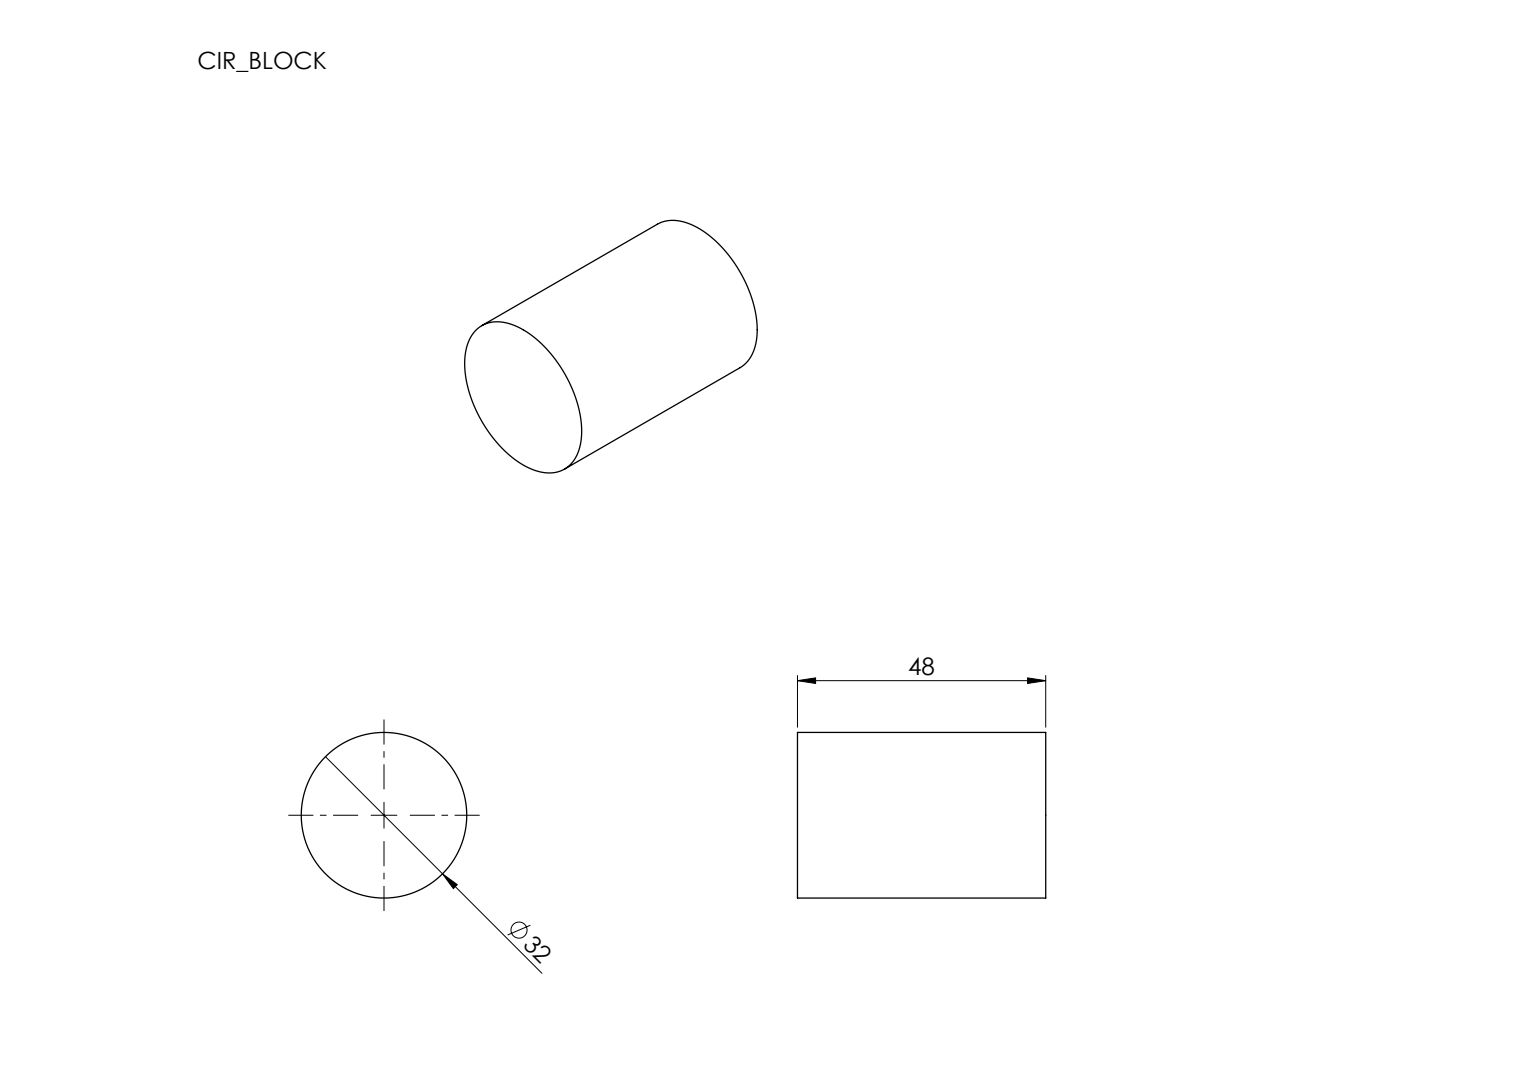
ISO-10303-21;
HEADER;
FILE_DESCRIPTION (('STEP AP214'),
    '1' );
FILE_NAME ('cir_block.step',
    '2026-10-08T13:22:57',
    ( '' ),
    ( '' ),
    'SwSTEP 2.0',
    'SolidWorks 2026',
    '' );
FILE_SCHEMA (( 'AUTOMOTIVE_DESIGN' ));
ENDSEC;

DATA;
#31=CARTESIAN_POINT ( 'NONE',  ( 0.000000000000000000, -6.162975822039154730E-30, 20.00000000000001776 ) ) ;
#245=CARTESIAN_POINT ( 'NONE',  ( 0.000000000000000000, 0.000000000000000000, 0.000000000000000000 ) ) ;
#365=( LENGTH_UNIT ( ) NAMED_UNIT ( * ) SI_UNIT ( .MILLI., .METRE. ) );
#415=( NAMED_UNIT ( * ) SI_UNIT ( $, .STERADIAN. ) SOLID_ANGLE_UNIT ( ) );
#499=AXIS2_PLACEMENT_3D ( 'NONE', #9498, #7831, #2505 ) ;
#736=DIRECTION ( 'NONE',  ( 0.000000000000000000, 0.000000000000000000, 1.000000000000000000 ) ) ;
#821=ORIENTED_EDGE ( 'NONE', *, *, #1366, .T. ) ;
#931=CYLINDRICAL_SURFACE ( 'NONE', #9784, 16.00000000000000000 ) ;
#1013=AXIS2_PLACEMENT_3D ( 'NONE', #4039, #3151, #6292 ) ;
#1129=ORIENTED_EDGE ( 'NONE', *, *, #9823, .F. ) ;
#1366=EDGE_CURVE ( 'NONE', #7651, #3104, #9591, .T. ) ;
#1410=SURFACE_SIDE_STYLE ('',( #7076 ) ) ;
#1441=COLOUR_RGB ( '', 0.08235294, 0.09019608, 0.10196078) ;
#1635=EDGE_LOOP ( 'NONE', ( #7592, #4013, #4601, #9629 ) ) ;
#1651=VERTEX_POINT ( 'NONE', #9037 ) ;
#1743=UNCERTAINTY_MEASURE_WITH_UNIT (LENGTH_MEASURE( 1.000000000000000082E-05 ), #365, 'distance_accuracy_value', 'NONE');
#1806=ADVANCED_FACE ( 'NONE', ( #7936 ), #3077, .F. ) ;
#1865=VECTOR ( 'NONE', #9017, 1000.000000000000000 ) ;
#1959=ORIENTED_EDGE ( 'NONE', *, *, #1366, .F. ) ;
#2023=CARTESIAN_POINT ( 'NONE',  ( 0.000000000000000000, -6.162975822039154730E-30, 20.00000000000001776 ) ) ;
#2058=PRODUCT_CONTEXT ( 'NONE', #2562, 'mechanical' ) ;
#2064=PRESENTATION_STYLE_ASSIGNMENT (( #4390 ) ) ;
#2281=SHAPE_REPRESENTATION_RELATIONSHIP ( 'NONE' , 'NONE' ,  #6629, #4260 ) ;
#2333=( LENGTH_UNIT ( ) NAMED_UNIT ( * ) SI_UNIT ( .MILLI., .METRE. ) );
#2443=ORIENTED_EDGE ( 'NONE', *, *, #5713, .T. ) ;
#2496=AXIS2_PLACEMENT_3D ( 'NONE', #9083, #5094, #6626 ) ;
#2505=DIRECTION ( 'NONE',  ( 0.000000000000000000, 1.000000000000000000, 0.000000000000000000 ) ) ;
#2562=APPLICATION_CONTEXT ( 'automotive_design' ) ;
#2586=DIRECTION ( 'NONE',  ( -1.000000000000000000, 0.000000000000000000, 0.000000000000000000 ) ) ;
#2590=STYLED_ITEM ( 'NONE', ( #2064 ), #3605 ) ;
#2631=DIRECTION ( 'NONE',  ( -0.000000000000000000, 0.000000000000000000, -1.000000000000000000 ) ) ;
#2728=SURFACE_STYLE_FILL_AREA ( #9781 ) ;
#2755=DIRECTION ( 'NONE',  ( -0.000000000000000000, 0.000000000000000000, -1.000000000000000000 ) ) ;
#2834=( NAMED_UNIT ( * ) PLANE_ANGLE_UNIT ( ) SI_UNIT ( $, .RADIAN. ) );
#2966=CARTESIAN_POINT ( 'NONE',  ( -16.00000000000000000, 0.000000000000000000, 68.00000000000000000 ) ) ;
#3077=PLANE ( 'NONE',  #6439 ) ;
#3102=FILL_AREA_STYLE ('',( #10087 ) ) ;
#3103=( GEOMETRIC_REPRESENTATION_CONTEXT ( 3 ) GLOBAL_UNCERTAINTY_ASSIGNED_CONTEXT ( ( #6479 ) ) GLOBAL_UNIT_ASSIGNED_CONTEXT ( ( #5379, #9370, #4709 ) ) REPRESENTATION_CONTEXT ( 'NONE', 'WORKASPACE' ) );
#3104=VERTEX_POINT ( 'NONE', #4823 ) ;
#3138=EDGE_LOOP ( 'NONE', ( #1959, #7031 ) ) ;
#3151=DIRECTION ( 'NONE',  ( 0.000000000000000000, 1.387778780781445676E-16, -1.000000000000000000 ) ) ;
#3185=DIRECTION ( 'NONE',  ( 0.000000000000000000, 0.000000000000000000, 1.000000000000000000 ) ) ;
#3249=FACE_OUTER_BOUND ( 'NONE', #10102, .T. ) ;
#3283=APPLICATION_CONTEXT ( 'automotive_design' ) ;
#3307=PLANE ( 'NONE',  #1013 ) ;
#3365=CYLINDRICAL_SURFACE ( 'NONE', #9653, 16.00000000000000000 ) ;
#3514=SURFACE_SIDE_STYLE ('',( #2728 ) ) ;
#3516=CARTESIAN_POINT ( 'NONE',  ( -16.00000000000000000, 0.000000000000000000, 113.2548339959390518 ) ) ;
#3605=MANIFOLD_SOLID_BREP ( 'Boss-Extrude1', #4495 ) ;
#3812=DIRECTION ( 'NONE',  ( 1.000000000000000000, 0.000000000000000000, 0.000000000000000000 ) ) ;
#3884=DIRECTION ( 'NONE',  ( 1.000000000000000000, 0.000000000000000000, 0.000000000000000000 ) ) ;
#3995=AXIS2_PLACEMENT_3D ( 'NONE', #245, #8930, #7419 ) ;
#4013=ORIENTED_EDGE ( 'NONE', *, *, #10208, .T. ) ;
#4021=PRODUCT_DEFINITION_CONTEXT ( 'detailed design', #3283, 'design' ) ;
#4039=CARTESIAN_POINT ( 'NONE',  ( 0.000000000000000000, 1.221245327087672352E-14, 68.00000000000000000 ) ) ;
#4050=EDGE_LOOP ( 'NONE', ( #1129, #5484 ) ) ;
#4095=STYLED_ITEM ( 'NONE', ( #7763 ), #4260 ) ;
#4103=PRODUCT_DEFINITION_FORMATION_WITH_SPECIFIED_SOURCE ( 'ANY', '', #7568, .NOT_KNOWN. ) ;
#4260=ADVANCED_BREP_SHAPE_REPRESENTATION ( '', ( #3605, #3995 ), #8889 ) ;
#4310=CIRCLE ( 'NONE', #2496, 16.00000000000000000 ) ;
#4320=UNCERTAINTY_MEASURE_WITH_UNIT (LENGTH_MEASURE( 1.000000000000000082E-05 ), #2333, 'distance_accuracy_value', 'NONE');
#4374=ADVANCED_FACE ( 'NONE', ( #3249 ), #931, .T. ) ;
#4390=SURFACE_STYLE_USAGE ( .BOTH. , #3514 ) ;
#4427=MECHANICAL_DESIGN_GEOMETRIC_PRESENTATION_REPRESENTATION('',(#4095),#3103);
#4495=CLOSED_SHELL ( 'NONE', ( #4374, #1806, #6248, #9894 ) ) ;
#4601=ORIENTED_EDGE ( 'NONE', *, *, #6775, .T. ) ;
#4709=( NAMED_UNIT ( * ) SI_UNIT ( $, .STERADIAN. ) SOLID_ANGLE_UNIT ( ) );
#4823=CARTESIAN_POINT ( 'NONE',  ( 16.00000000000000000, 1.959434878635765131E-15, 68.00000000000000000 ) ) ;
#5018=VECTOR ( 'NONE', #7541, 1000.000000000000000 ) ;
#5094=DIRECTION ( 'NONE',  ( 0.000000000000000000, 1.387778780781445676E-16, -1.000000000000000000 ) ) ;
#5181=DIRECTION ( 'NONE',  ( 0.000000000000000000, 0.000000000000000000, 1.000000000000000000 ) ) ;
#5379=( LENGTH_UNIT ( ) NAMED_UNIT ( * ) SI_UNIT ( .MILLI., .METRE. ) );
#5484=ORIENTED_EDGE ( 'NONE', *, *, #5776, .F. ) ;
#5702=ORIENTED_EDGE ( 'NONE', *, *, #6775, .F. ) ;
#5713=EDGE_CURVE ( 'NONE', #3104, #9748, #7610, .T. ) ;
#5776=EDGE_CURVE ( 'NONE', #9748, #1651, #8973, .T. ) ;
#5812=AXIS2_PLACEMENT_3D ( 'NONE', #2023, #5181, #9171 ) ;
#5900=DIRECTION ( 'NONE',  ( -1.000000000000000000, 0.000000000000000000, 0.000000000000000000 ) ) ;
#6242=( NAMED_UNIT ( * ) SI_UNIT ( $, .STERADIAN. ) SOLID_ANGLE_UNIT ( ) );
#6248=ADVANCED_FACE ( 'NONE', ( #8853 ), #3365, .T. ) ;
#6292=DIRECTION ( 'NONE',  ( -1.000000000000000000, 0.000000000000000000, 0.000000000000000000 ) ) ;
#6437=ORIENTED_EDGE ( 'NONE', *, *, #5776, .T. ) ;
#6439=AXIS2_PLACEMENT_3D ( 'NONE', #31, #3185, #3812 ) ;
#6442=CARTESIAN_POINT ( 'NONE',  ( 0.000000000000000000, 0.000000000000000000, 113.2548339959390518 ) ) ;
#6479=UNCERTAINTY_MEASURE_WITH_UNIT (LENGTH_MEASURE( 1.000000000000000082E-05 ), #5379, 'distance_accuracy_value', 'NONE');
#6626=DIRECTION ( 'NONE',  ( 0.000000000000000000, 1.000000000000000000, 0.000000000000000000 ) ) ;
#6629=SHAPE_REPRESENTATION ( 'cir_block', ( #3995 ), #8889 ) ;
#6775=EDGE_CURVE ( 'NONE', #7651, #1651, #9053, .T. ) ;
#6848=SHAPE_DEFINITION_REPRESENTATION ( #8218, #6629 ) ;
#6913=CARTESIAN_POINT ( 'NONE',  ( 16.00000000000000000, 1.959434878635765131E-15, 20.00000000000001776 ) ) ;
#6915=( NAMED_UNIT ( * ) PLANE_ANGLE_UNIT ( ) SI_UNIT ( $, .RADIAN. ) );
#7031=ORIENTED_EDGE ( 'NONE', *, *, #10208, .F. ) ;
#7076=SURFACE_STYLE_FILL_AREA ( #3102 ) ;
#7378=( GEOMETRIC_REPRESENTATION_CONTEXT ( 3 ) GLOBAL_UNCERTAINTY_ASSIGNED_CONTEXT ( ( #1743 ) ) GLOBAL_UNIT_ASSIGNED_CONTEXT ( ( #365, #2834, #415 ) ) REPRESENTATION_CONTEXT ( 'NONE', 'WORKASPACE' ) );
#7419=DIRECTION ( 'NONE',  ( 1.000000000000000000, 0.000000000000000000, 0.000000000000000000 ) ) ;
#7541=DIRECTION ( 'NONE',  ( -0.000000000000000000, 0.000000000000000000, -1.000000000000000000 ) ) ;
#7554=COLOUR_RGB ( '', 0.08235294, 0.09019608, 0.10196078) ;
#7568=PRODUCT ( 'cir_block', 'cir_block', '', ( #2058 ) ) ;
#7592=ORIENTED_EDGE ( 'NONE', *, *, #5713, .F. ) ;
#7610=LINE ( 'NONE', #8379, #1865 ) ;
#7651=VERTEX_POINT ( 'NONE', #2966 ) ;
#7763=PRESENTATION_STYLE_ASSIGNMENT (( #9320 ) ) ;
#7811=CARTESIAN_POINT ( 'NONE',  ( 0.000000000000000000, -6.162975822039154730E-30, 20.00000000000001776 ) ) ;
#7831=DIRECTION ( 'NONE',  ( 0.000000000000000000, 1.387778780781445676E-16, -1.000000000000000000 ) ) ;
#7936=FACE_OUTER_BOUND ( 'NONE', #4050, .T. ) ;
#8108=AXIS2_PLACEMENT_3D ( 'NONE', #7811, #736, #3884 ) ;
#8117=CARTESIAN_POINT ( 'NONE',  ( 0.000000000000000000, 0.000000000000000000, 113.2548339959390518 ) ) ;
#8208=FILL_AREA_STYLE_COLOUR ( '', #1441 ) ;
#8218=PRODUCT_DEFINITION_SHAPE ( 'NONE', 'NONE',  #8652 ) ;
#8379=CARTESIAN_POINT ( 'NONE',  ( 16.00000000000000000, 1.959434878635765131E-15, 113.2548339959390518 ) ) ;
#8652=PRODUCT_DEFINITION ( 'UNKNOWN', '', #4103, #4021 ) ;
#8688=FACE_OUTER_BOUND ( 'NONE', #3138, .T. ) ;
#8765=CIRCLE ( 'NONE', #8108, 16.00000000000000000 ) ;
#8853=FACE_OUTER_BOUND ( 'NONE', #1635, .T. ) ;
#8889=( GEOMETRIC_REPRESENTATION_CONTEXT ( 3 ) GLOBAL_UNCERTAINTY_ASSIGNED_CONTEXT ( ( #4320 ) ) GLOBAL_UNIT_ASSIGNED_CONTEXT ( ( #2333, #6915, #6242 ) ) REPRESENTATION_CONTEXT ( 'NONE', 'WORKASPACE' ) );
#8930=DIRECTION ( 'NONE',  ( 0.000000000000000000, 0.000000000000000000, 1.000000000000000000 ) ) ;
#8973=CIRCLE ( 'NONE', #5812, 16.00000000000000000 ) ;
#9017=DIRECTION ( 'NONE',  ( -0.000000000000000000, 0.000000000000000000, -1.000000000000000000 ) ) ;
#9037=CARTESIAN_POINT ( 'NONE',  ( -16.00000000000000000, 0.000000000000000000, 20.00000000000001776 ) ) ;
#9053=LINE ( 'NONE', #3516, #5018 ) ;
#9083=CARTESIAN_POINT ( 'NONE',  ( 0.000000000000000000, 0.000000000000000000, 68.00000000000000000 ) ) ;
#9171=DIRECTION ( 'NONE',  ( 1.000000000000000000, 0.000000000000000000, 0.000000000000000000 ) ) ;
#9320=SURFACE_STYLE_USAGE ( .BOTH. , #1410 ) ;
#9370=( NAMED_UNIT ( * ) PLANE_ANGLE_UNIT ( ) SI_UNIT ( $, .RADIAN. ) );
#9498=CARTESIAN_POINT ( 'NONE',  ( 0.000000000000000000, 0.000000000000000000, 68.00000000000000000 ) ) ;
#9591=CIRCLE ( 'NONE', #499, 16.00000000000000000 ) ;
#9629=ORIENTED_EDGE ( 'NONE', *, *, #9823, .T. ) ;
#9653=AXIS2_PLACEMENT_3D ( 'NONE', #8117, #2631, #2586 ) ;
#9696=MECHANICAL_DESIGN_GEOMETRIC_PRESENTATION_REPRESENTATION('',(#2590),#7378);
#9748=VERTEX_POINT ( 'NONE', #6913 ) ;
#9781=FILL_AREA_STYLE ('',( #8208 ) ) ;
#9784=AXIS2_PLACEMENT_3D ( 'NONE', #6442, #2755, #5900 ) ;
#9823=EDGE_CURVE ( 'NONE', #1651, #9748, #8765, .T. ) ;
#9894=ADVANCED_FACE ( 'NONE', ( #8688 ), #3307, .F. ) ;
#10087=FILL_AREA_STYLE_COLOUR ( '', #7554 ) ;
#10102=EDGE_LOOP ( 'NONE', ( #821, #2443, #6437, #5702 ) ) ;
#10208=EDGE_CURVE ( 'NONE', #3104, #7651, #4310, .T. ) ;
ENDSEC;
END-ISO-10303-21;
